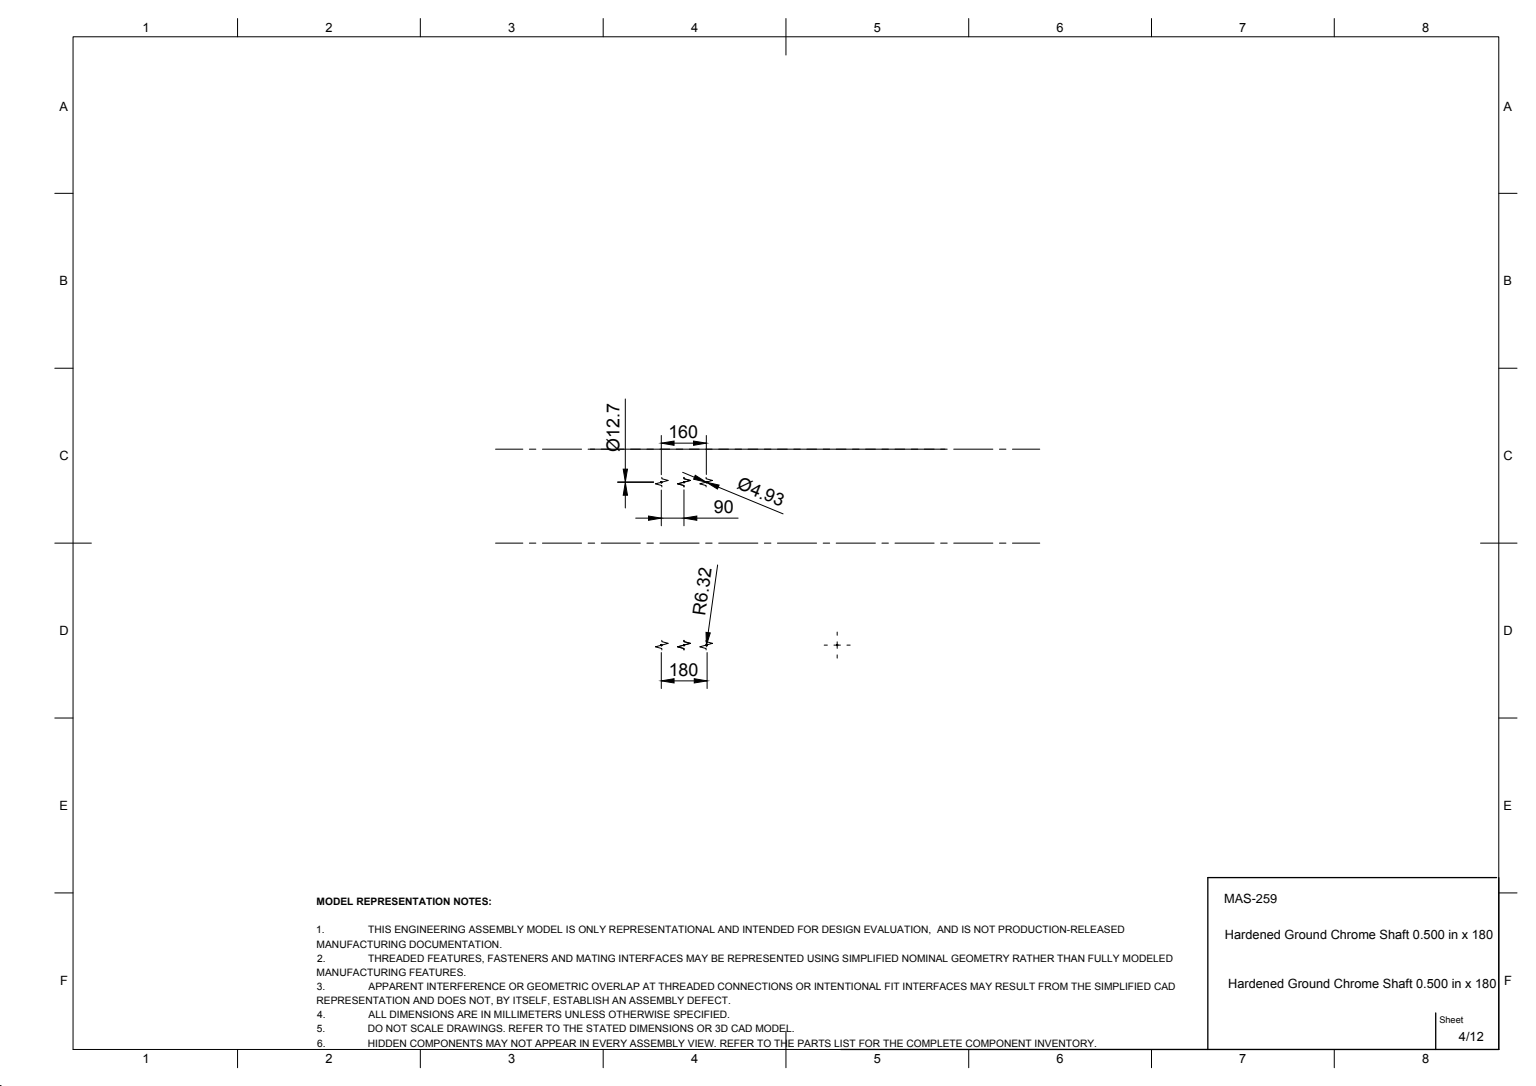
ISO-10303-21;
HEADER;
/* Generated by software containing ST-Developer
 * from STEP Tools, Inc. (www.steptools.com) 
 */

FILE_DESCRIPTION(
/* description */ (''),
/* implementation_level */ '2;1');

FILE_NAME(
/* name */ 'Hardened Ground Chrome Shaft 0.500 in x 180.step',
/* time_stamp */ '2026-10-15T13:30:17-07:00',
/* author */ (''),
/* organization */ (''),
/* preprocessor_version */ 'ST-DEVELOPER v20.2',
/* originating_system */ 'Autodesk Translation Framework v15.15.0.0',
/* authorisation */ '');

FILE_SCHEMA (('AUTOMOTIVE_DESIGN { 1 0 10303 214 3 1 1 }'));
ENDSEC;

DATA;
#10=MECHANICAL_DESIGN_GEOMETRIC_PRESENTATION_REPRESENTATION('',(#1035),#71795);
#1015=SHAPE_REPRESENTATION_RELATIONSHIP('SRR','None',#72019,#1025);
#1025=ADVANCED_BREP_SHAPE_REPRESENTATION('',(#1045),#71787);
#1035=STYLED_ITEM('',(#72078),#1045);
#1045=MANIFOLD_SOLID_BREP('Body1',#13637);
#1081=CONICAL_SURFACE('',#13996,2.464,1.02395598729616);
#1082=CONICAL_SURFACE('',#13999,2.464,1.02395598729616);
#1083=CONICAL_SURFACE('',#14002,2.464,1.02395598729616);
#1084=CONICAL_SURFACE('',#14005,6.1,0.785398163397447);
#1085=CONICAL_SURFACE('',#14009,6.1,0.785398163397439);
#1131=B_SPLINE_CURVE_WITH_KNOTS('',3,(#19389,#19390,#19391,#19392,#19393,
#19394,#19395,#19396,#19397,#19398,#19399,#19400,#19401,#19402,#19403,#19404,
#19405,#19406),.UNSPECIFIED.,.F.,.F.,(4,2,2,2,2,2,2,2,4),(0.,0.0939363144605702,
0.18787262892114,0.281725618013245,0.37557860710535,0.469431596197455,0.563284585289559,
0.657220899750131,0.751157214210703),.UNSPECIFIED.);
#1132=B_SPLINE_CURVE_WITH_KNOTS('',3,(#19407,#19408,#19409,#19410,#19411,
#19412,#19413,#19414,#19415,#19416,#19417,#19418,#19419,#19420,#19421,#19422,
#19423,#19424),.UNSPECIFIED.,.F.,.F.,(4,2,2,2,2,2,2,2,4),(0.751157214210703,
0.845093528671274,0.939029843131846,1.03288283222395,1.12673582131605,1.22058881040816,
1.31444179950026,1.40837811396083,1.50231442842141),.UNSPECIFIED.);
#1133=B_SPLINE_CURVE_WITH_KNOTS('',3,(#19434,#19435,#19436,#19437,#19438,
#19439,#19440,#19441,#19442,#19443,#19444,#19445,#19446,#19447,#19448,#19449,
#19450,#19451),.UNSPECIFIED.,.F.,.F.,(4,2,2,2,2,2,2,2,4),(0.,0.0939363144605709,
0.187872628921142,0.281725618013246,0.375578607105351,0.469431596197456,
0.56328458528956,0.657220899750131,0.751157214210702),.UNSPECIFIED.);
#1134=B_SPLINE_CURVE_WITH_KNOTS('',3,(#19452,#19453,#19454,#19455,#19456,
#19457,#19458,#19459,#19460,#19461,#19462,#19463,#19464,#19465,#19466,#19467,
#19468,#19469),.UNSPECIFIED.,.F.,.F.,(4,2,2,2,2,2,2,2,4),(0.751157214210702,
0.845093528671273,0.939029843131844,1.03288283222395,1.12673582131605,1.22058881040816,
1.31444179950026,1.40837811396083,1.5023144284214),.UNSPECIFIED.);
#1135=B_SPLINE_CURVE_WITH_KNOTS('',3,(#19479,#19480,#19481,#19482,#19483,
#19484,#19485,#19486,#19487,#19488,#19489,#19490,#19491,#19492,#19493,#19494,
#19495,#19496),.UNSPECIFIED.,.F.,.F.,(4,2,2,2,2,2,2,2,4),(0.,0.0939363144605713,
0.187872628921143,0.281725618013247,0.375578607105351,0.469431596197456,
0.56328458528956,0.657220899750132,0.751157214210703),.UNSPECIFIED.);
#1136=B_SPLINE_CURVE_WITH_KNOTS('',3,(#19497,#19498,#19499,#19500,#19501,
#19502,#19503,#19504,#19505,#19506,#19507,#19508,#19509,#19510,#19511,#19512,
#19513,#19514),.UNSPECIFIED.,.F.,.F.,(4,2,2,2,2,2,2,2,4),(0.751157214210703,
0.845093528671273,0.939029843131844,1.03288283222395,1.12673582131605,1.22058881040816,
1.31444179950026,1.40837811396083,1.5023144284214),.UNSPECIFIED.);
#1542=FACE_BOUND('',#2862,.T.);
#1543=FACE_BOUND('',#2863,.T.);
#1544=FACE_BOUND('',#2864,.T.);
#1611=PLANE('',#14003);
#1612=PLANE('',#14011);
#2147=FACE_OUTER_BOUND('',#2853,.T.);
#2148=FACE_OUTER_BOUND('',#2854,.T.);
#2149=FACE_OUTER_BOUND('',#2855,.T.);
#2150=FACE_OUTER_BOUND('',#2856,.T.);
#2151=FACE_OUTER_BOUND('',#2857,.T.);
#2152=FACE_OUTER_BOUND('',#2858,.T.);
#2153=FACE_OUTER_BOUND('',#2859,.T.);
#2154=FACE_OUTER_BOUND('',#2860,.T.);
#2155=FACE_OUTER_BOUND('',#2861,.T.);
#2156=FACE_OUTER_BOUND('',#2865,.T.);
#2157=FACE_OUTER_BOUND('',#2866,.T.);
#2853=EDGE_LOOP('',(#9525,#9526,#9527,#9528,#9529));
#2854=EDGE_LOOP('',(#9530,#9531,#9532));
#2855=EDGE_LOOP('',(#9533,#9534,#9535,#9536,#9537));
#2856=EDGE_LOOP('',(#9538,#9539,#9540));
#2857=EDGE_LOOP('',(#9541,#9542,#9543,#9544,#9545));
#2858=EDGE_LOOP('',(#9546,#9547,#9548));
#2859=EDGE_LOOP('',(#9549));
#2860=EDGE_LOOP('',(#9550,#9551,#9552,#9553));
#2861=EDGE_LOOP('',(#9554,#9555,#9556,#9557));
#2862=EDGE_LOOP('',(#9558,#9559));
#2863=EDGE_LOOP('',(#9560,#9561));
#2864=EDGE_LOOP('',(#9562,#9563));
#2865=EDGE_LOOP('',(#9564,#9565,#9566,#9567));
#2866=EDGE_LOOP('',(#9568));
#3512=CIRCLE('',#13995,2.464);
#3513=CIRCLE('',#13998,2.464);
#3514=CIRCLE('',#14001,2.464);
#3515=CIRCLE('',#14004,5.85);
#3516=CIRCLE('',#14006,6.35);
#3517=CIRCLE('',#14008,6.35);
#3518=CIRCLE('',#14010,5.85);
#3976=LINE('',#19426,#4887);
#3977=LINE('',#19430,#4888);
#3978=LINE('',#19471,#4889);
#3979=LINE('',#19475,#4890);
#3980=LINE('',#19516,#4891);
#3981=LINE('',#19520,#4892);
#3982=LINE('',#19527,#4893);
#3983=LINE('',#19531,#4894);
#3984=LINE('',#19534,#4895);
#4887=VECTOR('',#15659,2.464);
#4888=VECTOR('',#15664,2.464);
#4889=VECTOR('',#15667,2.464);
#4890=VECTOR('',#15672,2.464);
#4891=VECTOR('',#15675,2.464);
#4892=VECTOR('',#15680,2.464);
#4893=VECTOR('',#15689,6.1);
#4894=VECTOR('',#15694,6.35);
#4895=VECTOR('',#15697,6.1);
#5852=VERTEX_POINT('',#19387);
#5853=VERTEX_POINT('',#19388);
#5854=VERTEX_POINT('',#19425);
#5855=VERTEX_POINT('',#19429);
#5856=VERTEX_POINT('',#19432);
#5857=VERTEX_POINT('',#19433);
#5858=VERTEX_POINT('',#19470);
#5859=VERTEX_POINT('',#19474);
#5860=VERTEX_POINT('',#19477);
#5861=VERTEX_POINT('',#19478);
#5862=VERTEX_POINT('',#19515);
#5863=VERTEX_POINT('',#19519);
#5864=VERTEX_POINT('',#19522);
#5865=VERTEX_POINT('',#19525);
#5866=VERTEX_POINT('',#19529);
#5867=VERTEX_POINT('',#19533);
#7297=EDGE_CURVE('',#5852,#5853,#1131,.T.);
#7298=EDGE_CURVE('',#5853,#5852,#1132,.T.);
#7299=EDGE_CURVE('',#5853,#5854,#3976,.T.);
#7300=EDGE_CURVE('',#5854,#5854,#3512,.T.);
#7301=EDGE_CURVE('',#5855,#5854,#3977,.T.);
#7302=EDGE_CURVE('',#5856,#5857,#1133,.T.);
#7303=EDGE_CURVE('',#5857,#5856,#1134,.T.);
#7304=EDGE_CURVE('',#5857,#5858,#3978,.T.);
#7305=EDGE_CURVE('',#5858,#5858,#3513,.T.);
#7306=EDGE_CURVE('',#5859,#5858,#3979,.T.);
#7307=EDGE_CURVE('',#5860,#5861,#1135,.T.);
#7308=EDGE_CURVE('',#5861,#5860,#1136,.T.);
#7309=EDGE_CURVE('',#5861,#5862,#3980,.T.);
#7310=EDGE_CURVE('',#5862,#5862,#3514,.T.);
#7311=EDGE_CURVE('',#5863,#5862,#3981,.T.);
#7312=EDGE_CURVE('',#5864,#5864,#3515,.T.);
#7313=EDGE_CURVE('',#5865,#5865,#3516,.T.);
#7314=EDGE_CURVE('',#5865,#5864,#3982,.T.);
#7315=EDGE_CURVE('',#5866,#5866,#3517,.T.);
#7316=EDGE_CURVE('',#5866,#5865,#3983,.T.);
#7317=EDGE_CURVE('',#5866,#5867,#3984,.T.);
#7318=EDGE_CURVE('',#5867,#5867,#3518,.T.);
#9525=ORIENTED_EDGE('',*,*,#7297,.F.);
#9526=ORIENTED_EDGE('',*,*,#7298,.F.);
#9527=ORIENTED_EDGE('',*,*,#7299,.T.);
#9528=ORIENTED_EDGE('',*,*,#7300,.T.);
#9529=ORIENTED_EDGE('',*,*,#7299,.F.);
#9530=ORIENTED_EDGE('',*,*,#7301,.T.);
#9531=ORIENTED_EDGE('',*,*,#7300,.F.);
#9532=ORIENTED_EDGE('',*,*,#7301,.F.);
#9533=ORIENTED_EDGE('',*,*,#7302,.F.);
#9534=ORIENTED_EDGE('',*,*,#7303,.F.);
#9535=ORIENTED_EDGE('',*,*,#7304,.T.);
#9536=ORIENTED_EDGE('',*,*,#7305,.T.);
#9537=ORIENTED_EDGE('',*,*,#7304,.F.);
#9538=ORIENTED_EDGE('',*,*,#7306,.T.);
#9539=ORIENTED_EDGE('',*,*,#7305,.F.);
#9540=ORIENTED_EDGE('',*,*,#7306,.F.);
#9541=ORIENTED_EDGE('',*,*,#7307,.F.);
#9542=ORIENTED_EDGE('',*,*,#7308,.F.);
#9543=ORIENTED_EDGE('',*,*,#7309,.T.);
#9544=ORIENTED_EDGE('',*,*,#7310,.T.);
#9545=ORIENTED_EDGE('',*,*,#7309,.F.);
#9546=ORIENTED_EDGE('',*,*,#7311,.T.);
#9547=ORIENTED_EDGE('',*,*,#7310,.F.);
#9548=ORIENTED_EDGE('',*,*,#7311,.F.);
#9549=ORIENTED_EDGE('',*,*,#7312,.F.);
#9550=ORIENTED_EDGE('',*,*,#7313,.F.);
#9551=ORIENTED_EDGE('',*,*,#7314,.T.);
#9552=ORIENTED_EDGE('',*,*,#7312,.T.);
#9553=ORIENTED_EDGE('',*,*,#7314,.F.);
#9554=ORIENTED_EDGE('',*,*,#7315,.F.);
#9555=ORIENTED_EDGE('',*,*,#7316,.T.);
#9556=ORIENTED_EDGE('',*,*,#7313,.T.);
#9557=ORIENTED_EDGE('',*,*,#7316,.F.);
#9558=ORIENTED_EDGE('',*,*,#7297,.T.);
#9559=ORIENTED_EDGE('',*,*,#7298,.T.);
#9560=ORIENTED_EDGE('',*,*,#7302,.T.);
#9561=ORIENTED_EDGE('',*,*,#7303,.T.);
#9562=ORIENTED_EDGE('',*,*,#7307,.T.);
#9563=ORIENTED_EDGE('',*,*,#7308,.T.);
#9564=ORIENTED_EDGE('',*,*,#7315,.T.);
#9565=ORIENTED_EDGE('',*,*,#7317,.T.);
#9566=ORIENTED_EDGE('',*,*,#7318,.F.);
#9567=ORIENTED_EDGE('',*,*,#7317,.F.);
#9568=ORIENTED_EDGE('',*,*,#7318,.T.);
#12907=CYLINDRICAL_SURFACE('',#13994,2.464);
#12908=CYLINDRICAL_SURFACE('',#13997,2.464);
#12909=CYLINDRICAL_SURFACE('',#14000,2.464);
#12910=CYLINDRICAL_SURFACE('',#14007,6.35);
#13107=ADVANCED_FACE('',(#2147),#12907,.F.);
#13108=ADVANCED_FACE('',(#2148),#1081,.F.);
#13109=ADVANCED_FACE('',(#2149),#12908,.F.);
#13110=ADVANCED_FACE('',(#2150),#1082,.F.);
#13111=ADVANCED_FACE('',(#2151),#12909,.F.);
#13112=ADVANCED_FACE('',(#2152),#1083,.F.);
#13113=ADVANCED_FACE('',(#2153),#1611,.T.);
#13114=ADVANCED_FACE('',(#2154),#1084,.T.);
#13115=ADVANCED_FACE('',(#2155,#1542,#1543,#1544),#12910,.T.);
#13116=ADVANCED_FACE('',(#2156),#1085,.T.);
#13117=ADVANCED_FACE('',(#2157),#1612,.T.);
#13637=CLOSED_SHELL('',(#13107,#13108,#13109,#13110,#13111,#13112,#13113,
#13114,#13115,#13116,#13117));
#13993=AXIS2_PLACEMENT_3D('',#19385,#15655,#15656);
#13994=AXIS2_PLACEMENT_3D('',#19386,#15657,#15658);
#13995=AXIS2_PLACEMENT_3D('',#19427,#15660,#15661);
#13996=AXIS2_PLACEMENT_3D('',#19428,#15662,#15663);
#13997=AXIS2_PLACEMENT_3D('',#19431,#15665,#15666);
#13998=AXIS2_PLACEMENT_3D('',#19472,#15668,#15669);
#13999=AXIS2_PLACEMENT_3D('',#19473,#15670,#15671);
#14000=AXIS2_PLACEMENT_3D('',#19476,#15673,#15674);
#14001=AXIS2_PLACEMENT_3D('',#19517,#15676,#15677);
#14002=AXIS2_PLACEMENT_3D('',#19518,#15678,#15679);
#14003=AXIS2_PLACEMENT_3D('',#19521,#15681,#15682);
#14004=AXIS2_PLACEMENT_3D('',#19523,#15683,#15684);
#14005=AXIS2_PLACEMENT_3D('',#19524,#15685,#15686);
#14006=AXIS2_PLACEMENT_3D('',#19526,#15687,#15688);
#14007=AXIS2_PLACEMENT_3D('',#19528,#15690,#15691);
#14008=AXIS2_PLACEMENT_3D('',#19530,#15692,#15693);
#14009=AXIS2_PLACEMENT_3D('',#19532,#15695,#15696);
#14010=AXIS2_PLACEMENT_3D('',#19535,#15698,#15699);
#14011=AXIS2_PLACEMENT_3D('',#19536,#15700,#15701);
#15655=DIRECTION('axis',(0.,0.,1.));
#15656=DIRECTION('refdir',(1.,0.,0.));
#15657=DIRECTION('center_axis',(0.,0.707106781186548,0.707106781186548));
#15658=DIRECTION('ref_axis',(0.,-0.707106781186548,0.707106781186548));
#15659=DIRECTION('',(0.,0.707106781186548,0.707106781186548));
#15660=DIRECTION('center_axis',(0.,0.707106781186548,0.707106781186548));
#15661=DIRECTION('ref_axis',(1.,0.,0.));
#15662=DIRECTION('center_axis',(0.,-0.707106781186548,-0.707106781186548));
#15663=DIRECTION('ref_axis',(0.,-0.707106781186548,0.707106781186548));
#15664=DIRECTION('',(1.04605873377251E-16,0.236301539303659,-0.971679773651135));
#15665=DIRECTION('center_axis',(0.,0.707106781186548,0.707106781186548));
#15666=DIRECTION('ref_axis',(0.,-0.707106781186548,0.707106781186548));
#15667=DIRECTION('',(0.,0.707106781186548,0.707106781186548));
#15668=DIRECTION('center_axis',(0.,0.707106781186548,0.707106781186548));
#15669=DIRECTION('ref_axis',(1.,0.,0.));
#15670=DIRECTION('center_axis',(0.,-0.707106781186548,-0.707106781186548));
#15671=DIRECTION('ref_axis',(0.,-0.707106781186548,0.707106781186548));
#15672=DIRECTION('',(1.04605873377251E-16,0.236301539303659,-0.971679773651135));
#15673=DIRECTION('center_axis',(0.,0.707106781186548,0.707106781186548));
#15674=DIRECTION('ref_axis',(0.,-0.707106781186548,0.707106781186548));
#15675=DIRECTION('',(0.,0.707106781186548,0.707106781186548));
#15676=DIRECTION('center_axis',(0.,0.707106781186548,0.707106781186548));
#15677=DIRECTION('ref_axis',(1.,0.,0.));
#15678=DIRECTION('center_axis',(0.,-0.707106781186548,-0.707106781186548));
#15679=DIRECTION('ref_axis',(0.,-0.707106781186548,0.707106781186548));
#15680=DIRECTION('',(1.04605873377251E-16,0.236301539303659,-0.971679773651135));
#15681=DIRECTION('center_axis',(-1.,0.,0.));
#15682=DIRECTION('ref_axis',(0.,0.,1.));
#15683=DIRECTION('center_axis',(1.,0.,0.));
#15684=DIRECTION('ref_axis',(0.,0.,-1.));
#15685=DIRECTION('center_axis',(1.,0.,0.));
#15686=DIRECTION('ref_axis',(0.,1.,0.));
#15687=DIRECTION('center_axis',(1.,0.,0.));
#15688=DIRECTION('ref_axis',(0.,0.,-1.));
#15689=DIRECTION('',(-0.707106781186548,0.707106781186547,8.65956056235492E-17));
#15690=DIRECTION('center_axis',(1.,0.,0.));
#15691=DIRECTION('ref_axis',(0.,1.,0.));
#15692=DIRECTION('center_axis',(1.,0.,0.));
#15693=DIRECTION('ref_axis',(0.,0.,-1.));
#15694=DIRECTION('',(-1.,0.,0.));
#15695=DIRECTION('center_axis',(-1.,0.,0.));
#15696=DIRECTION('ref_axis',(0.,1.,0.));
#15697=DIRECTION('',(0.707106781186554,0.707106781186541,-8.65956056235485E-17));
#15698=DIRECTION('center_axis',(1.,0.,0.));
#15699=DIRECTION('ref_axis',(0.,0.,-1.));
#15700=DIRECTION('center_axis',(1.,0.,0.));
#15701=DIRECTION('ref_axis',(0.,0.,-1.));
#19385=CARTESIAN_POINT('',(0.,0.,0.));
#19386=CARTESIAN_POINT('Origin',(160.,20.386522368915,36.261522368915));
#19387=CARTESIAN_POINT('',(160.,16.3443798161838,35.7040020338711));
#19388=CARTESIAN_POINT('',(160.,19.8290020338711,32.2193798161838));
#19389=CARTESIAN_POINT('Ctrl Pts',(160.,16.3443798161838,35.7040020338711));
#19390=CARTESIAN_POINT('Ctrl Pts',(160.313121048202,16.3443798161838,35.7040020338711));
#19391=CARTESIAN_POINT('Ctrl Pts',(160.644530562725,16.3694605042293,35.639628490954));
#19392=CARTESIAN_POINT('Ctrl Pts',(161.250438810992,16.4794607587991,35.3926861336962));
#19393=CARTESIAN_POINT('Ctrl Pts',(161.525274451059,16.5655176229446,35.2114538079158));
#19394=CARTESIAN_POINT('Ctrl Pts',(161.9591552462,16.7847783338415,34.8171144138708));
#19395=CARTESIAN_POINT('Ctrl Pts',(162.148303695899,16.9331965285742,34.5767521893323));
#19396=CARTESIAN_POINT('Ctrl Pts',(162.400811747278,17.2971590391485,34.083429001318));
#19397=CARTESIAN_POINT('Ctrl Pts',(162.464,17.5136583227266,33.8310855562043));
#19398=CARTESIAN_POINT('Ctrl Pts',(162.464,17.9560855562043,33.3886583227266));
#19399=CARTESIAN_POINT('Ctrl Pts',(162.400811747278,18.208429001318,33.1721590391485));
#19400=CARTESIAN_POINT('Ctrl Pts',(162.148303695899,18.7017521893323,32.8081965285742));
#19401=CARTESIAN_POINT('Ctrl Pts',(161.9591552462,18.9421144138708,32.6597783338415));
#19402=CARTESIAN_POINT('Ctrl Pts',(161.525274451059,19.3364538079158,32.4405176229446));
#19403=CARTESIAN_POINT('Ctrl Pts',(161.250438810992,19.5176861336962,32.3544607587991));
#19404=CARTESIAN_POINT('Ctrl Pts',(160.644530562725,19.764628490954,32.2444605042293));
#19405=CARTESIAN_POINT('Ctrl Pts',(160.313121048202,19.8290020338711,32.2193798161838));
#19406=CARTESIAN_POINT('Ctrl Pts',(160.,19.8290020338711,32.2193798161838));
#19407=CARTESIAN_POINT('Ctrl Pts',(160.,19.8290020338711,32.2193798161838));
#19408=CARTESIAN_POINT('Ctrl Pts',(159.686878951798,19.8290020338711,32.2193798161838));
#19409=CARTESIAN_POINT('Ctrl Pts',(159.355469437275,19.764628490954,32.2444605042293));
#19410=CARTESIAN_POINT('Ctrl Pts',(158.749561189008,19.5176861336961,32.3544607587991));
#19411=CARTESIAN_POINT('Ctrl Pts',(158.474725548941,19.3364538079158,32.4405176229446));
#19412=CARTESIAN_POINT('Ctrl Pts',(158.0408447538,18.9421144138708,32.6597783338415));
#19413=CARTESIAN_POINT('Ctrl Pts',(157.851696304101,18.7017521893323,32.8081965285742));
#19414=CARTESIAN_POINT('Ctrl Pts',(157.599188252722,18.208429001318,33.1721590391485));
#19415=CARTESIAN_POINT('Ctrl Pts',(157.536,17.9560855562043,33.3886583227266));
#19416=CARTESIAN_POINT('Ctrl Pts',(157.536,17.5136583227266,33.8310855562043));
#19417=CARTESIAN_POINT('Ctrl Pts',(157.599188252722,17.2971590391485,34.083429001318));
#19418=CARTESIAN_POINT('Ctrl Pts',(157.851696304101,16.9331965285742,34.5767521893323));
#19419=CARTESIAN_POINT('Ctrl Pts',(158.0408447538,16.7847783338415,34.8171144138708));
#19420=CARTESIAN_POINT('Ctrl Pts',(158.474725548941,16.5655176229446,35.2114538079158));
#19421=CARTESIAN_POINT('Ctrl Pts',(158.749561189008,16.4794607587991,35.3926861336961));
#19422=CARTESIAN_POINT('Ctrl Pts',(159.355469437275,16.3694605042293,35.639628490954));
#19423=CARTESIAN_POINT('Ctrl Pts',(159.686878951798,16.3443798161838,35.7040020338711));
#19424=CARTESIAN_POINT('Ctrl Pts',(160.,16.3443798161838,35.7040020338711));
#19425=CARTESIAN_POINT('',(160.,25.1340372978015,37.5244150801141));
#19426=CARTESIAN_POINT('',(160.,22.1288334777587,34.5192112600714));
#19427=CARTESIAN_POINT('Origin',(160.,23.3917261889578,39.2667261889578));
#19428=CARTESIAN_POINT('Origin',(160.,23.3917261889578,39.2667261889578));
#19429=CARTESIAN_POINT('',(160.,24.4523863607376,40.3273863607376));
#19430=CARTESIAN_POINT('',(160.,25.1340372978015,37.5244150801141));
#19431=CARTESIAN_POINT('Origin',(90.,20.386522368915,36.261522368915));
#19432=CARTESIAN_POINT('',(90.,16.3443798161838,35.7040020338711));
#19433=CARTESIAN_POINT('',(90.,19.8290020338711,32.2193798161838));
#19434=CARTESIAN_POINT('Ctrl Pts',(90.,16.3443798161838,35.7040020338711));
#19435=CARTESIAN_POINT('Ctrl Pts',(90.3131210482019,16.3443798161838,35.7040020338711));
#19436=CARTESIAN_POINT('Ctrl Pts',(90.6445305627248,16.3694605042293,35.639628490954));
#19437=CARTESIAN_POINT('Ctrl Pts',(91.2504388109923,16.4794607587991,35.3926861336961));
#19438=CARTESIAN_POINT('Ctrl Pts',(91.525274451059,16.5655176229446,35.2114538079158));
#19439=CARTESIAN_POINT('Ctrl Pts',(91.9591552462002,16.7847783338415,34.8171144138708));
#19440=CARTESIAN_POINT('Ctrl Pts',(92.1483036958993,16.9331965285742,34.5767521893323));
#19441=CARTESIAN_POINT('Ctrl Pts',(92.4008117472775,17.2971590391485,34.0834290013181));
#19442=CARTESIAN_POINT('Ctrl Pts',(92.464,17.5136583227266,33.8310855562043));
#19443=CARTESIAN_POINT('Ctrl Pts',(92.464,17.9560855562043,33.3886583227266));
#19444=CARTESIAN_POINT('Ctrl Pts',(92.4008117472775,18.208429001318,33.1721590391485));
#19445=CARTESIAN_POINT('Ctrl Pts',(92.1483036958993,18.7017521893323,32.8081965285742));
#19446=CARTESIAN_POINT('Ctrl Pts',(91.9591552462002,18.9421144138708,32.6597783338415));
#19447=CARTESIAN_POINT('Ctrl Pts',(91.525274451059,19.3364538079158,32.4405176229446));
#19448=CARTESIAN_POINT('Ctrl Pts',(91.2504388109923,19.5176861336961,32.3544607587991));
#19449=CARTESIAN_POINT('Ctrl Pts',(90.6445305627248,19.764628490954,32.2444605042293));
#19450=CARTESIAN_POINT('Ctrl Pts',(90.3131210482019,19.8290020338711,32.2193798161838));
#19451=CARTESIAN_POINT('Ctrl Pts',(90.,19.8290020338711,32.2193798161838));
#19452=CARTESIAN_POINT('Ctrl Pts',(90.,19.8290020338711,32.2193798161838));
#19453=CARTESIAN_POINT('Ctrl Pts',(89.6868789517981,19.8290020338711,32.2193798161838));
#19454=CARTESIAN_POINT('Ctrl Pts',(89.3554694372752,19.764628490954,32.2444605042293));
#19455=CARTESIAN_POINT('Ctrl Pts',(88.7495611890077,19.5176861336961,32.3544607587991));
#19456=CARTESIAN_POINT('Ctrl Pts',(88.474725548941,19.3364538079158,32.4405176229446));
#19457=CARTESIAN_POINT('Ctrl Pts',(88.0408447537999,18.9421144138708,32.6597783338415));
#19458=CARTESIAN_POINT('Ctrl Pts',(87.8516963041007,18.7017521893323,32.8081965285742));
#19459=CARTESIAN_POINT('Ctrl Pts',(87.5991882527224,18.208429001318,33.1721590391485));
#19460=CARTESIAN_POINT('Ctrl Pts',(87.536,17.9560855562043,33.3886583227266));
#19461=CARTESIAN_POINT('Ctrl Pts',(87.536,17.5136583227266,33.8310855562043));
#19462=CARTESIAN_POINT('Ctrl Pts',(87.5991882527224,17.2971590391485,34.0834290013181));
#19463=CARTESIAN_POINT('Ctrl Pts',(87.8516963041007,16.9331965285742,34.5767521893323));
#19464=CARTESIAN_POINT('Ctrl Pts',(88.0408447537999,16.7847783338415,34.8171144138708));
#19465=CARTESIAN_POINT('Ctrl Pts',(88.474725548941,16.5655176229446,35.2114538079158));
#19466=CARTESIAN_POINT('Ctrl Pts',(88.7495611890077,16.4794607587991,35.3926861336961));
#19467=CARTESIAN_POINT('Ctrl Pts',(89.3554694372752,16.3694605042293,35.639628490954));
#19468=CARTESIAN_POINT('Ctrl Pts',(89.6868789517981,16.3443798161838,35.7040020338711));
#19469=CARTESIAN_POINT('Ctrl Pts',(90.,16.3443798161838,35.7040020338711));
#19470=CARTESIAN_POINT('',(90.,25.1340372978015,37.5244150801141));
#19471=CARTESIAN_POINT('',(90.,22.1288334777587,34.5192112600714));
#19472=CARTESIAN_POINT('Origin',(90.,23.3917261889578,39.2667261889578));
#19473=CARTESIAN_POINT('Origin',(90.,23.3917261889578,39.2667261889578));
#19474=CARTESIAN_POINT('',(90.,24.4523863607376,40.3273863607376));
#19475=CARTESIAN_POINT('',(90.,25.1340372978015,37.5244150801141));
#19476=CARTESIAN_POINT('Origin',(20.,20.386522368915,36.261522368915));
#19477=CARTESIAN_POINT('',(20.,16.3443798161838,35.7040020338711));
#19478=CARTESIAN_POINT('',(20.,19.8290020338711,32.2193798161838));
#19479=CARTESIAN_POINT('Ctrl Pts',(20.,16.3443798161838,35.7040020338711));
#19480=CARTESIAN_POINT('Ctrl Pts',(20.3131210482019,16.3443798161838,35.7040020338711));
#19481=CARTESIAN_POINT('Ctrl Pts',(20.6445305627248,16.3694605042293,35.639628490954));
#19482=CARTESIAN_POINT('Ctrl Pts',(21.2504388109924,16.4794607587991,35.3926861336961));
#19483=CARTESIAN_POINT('Ctrl Pts',(21.525274451059,16.5655176229446,35.2114538079158));
#19484=CARTESIAN_POINT('Ctrl Pts',(21.9591552462002,16.7847783338415,34.8171144138708));
#19485=CARTESIAN_POINT('Ctrl Pts',(22.1483036958993,16.9331965285742,34.5767521893323));
#19486=CARTESIAN_POINT('Ctrl Pts',(22.4008117472775,17.2971590391485,34.083429001318));
#19487=CARTESIAN_POINT('Ctrl Pts',(22.464,17.5136583227266,33.8310855562043));
#19488=CARTESIAN_POINT('Ctrl Pts',(22.464,17.9560855562043,33.3886583227266));
#19489=CARTESIAN_POINT('Ctrl Pts',(22.4008117472775,18.208429001318,33.1721590391485));
#19490=CARTESIAN_POINT('Ctrl Pts',(22.1483036958993,18.7017521893323,32.8081965285742));
#19491=CARTESIAN_POINT('Ctrl Pts',(21.9591552462002,18.9421144138708,32.6597783338415));
#19492=CARTESIAN_POINT('Ctrl Pts',(21.525274451059,19.3364538079158,32.4405176229446));
#19493=CARTESIAN_POINT('Ctrl Pts',(21.2504388109924,19.5176861336961,32.3544607587991));
#19494=CARTESIAN_POINT('Ctrl Pts',(20.6445305627248,19.764628490954,32.2444605042293));
#19495=CARTESIAN_POINT('Ctrl Pts',(20.3131210482019,19.8290020338711,32.2193798161838));
#19496=CARTESIAN_POINT('Ctrl Pts',(20.,19.8290020338711,32.2193798161838));
#19497=CARTESIAN_POINT('Ctrl Pts',(20.,19.8290020338711,32.2193798161838));
#19498=CARTESIAN_POINT('Ctrl Pts',(19.6868789517981,19.8290020338711,32.2193798161838));
#19499=CARTESIAN_POINT('Ctrl Pts',(19.3554694372752,19.764628490954,32.2444605042293));
#19500=CARTESIAN_POINT('Ctrl Pts',(18.7495611890077,19.5176861336961,32.3544607587991));
#19501=CARTESIAN_POINT('Ctrl Pts',(18.474725548941,19.3364538079158,32.4405176229446));
#19502=CARTESIAN_POINT('Ctrl Pts',(18.0408447537999,18.9421144138708,32.6597783338415));
#19503=CARTESIAN_POINT('Ctrl Pts',(17.8516963041007,18.7017521893323,32.8081965285742));
#19504=CARTESIAN_POINT('Ctrl Pts',(17.5991882527225,18.208429001318,33.1721590391485));
#19505=CARTESIAN_POINT('Ctrl Pts',(17.536,17.9560855562043,33.3886583227266));
#19506=CARTESIAN_POINT('Ctrl Pts',(17.536,17.5136583227266,33.8310855562043));
#19507=CARTESIAN_POINT('Ctrl Pts',(17.5991882527225,17.2971590391485,34.0834290013181));
#19508=CARTESIAN_POINT('Ctrl Pts',(17.8516963041007,16.9331965285742,34.5767521893323));
#19509=CARTESIAN_POINT('Ctrl Pts',(18.0408447537999,16.7847783338415,34.8171144138708));
#19510=CARTESIAN_POINT('Ctrl Pts',(18.474725548941,16.5655176229446,35.2114538079158));
#19511=CARTESIAN_POINT('Ctrl Pts',(18.7495611890077,16.4794607587991,35.3926861336961));
#19512=CARTESIAN_POINT('Ctrl Pts',(19.3554694372752,16.3694605042293,35.639628490954));
#19513=CARTESIAN_POINT('Ctrl Pts',(19.6868789517981,16.3443798161838,35.7040020338711));
#19514=CARTESIAN_POINT('Ctrl Pts',(20.,16.3443798161838,35.7040020338711));
#19515=CARTESIAN_POINT('',(20.,25.1340372978015,37.5244150801141));
#19516=CARTESIAN_POINT('',(20.,22.1288334777587,34.5192112600714));
#19517=CARTESIAN_POINT('Origin',(20.,23.3917261889578,39.2667261889578));
#19518=CARTESIAN_POINT('Origin',(20.,23.3917261889578,39.2667261889578));
#19519=CARTESIAN_POINT('',(20.,24.4523863607376,40.3273863607376));
#19520=CARTESIAN_POINT('',(20.,25.1340372978015,37.5244150801141));
#19521=CARTESIAN_POINT('Origin',(0.,28.075,38.1));
#19522=CARTESIAN_POINT('',(-7.25114412958305E-15,16.375,38.1));
#19523=CARTESIAN_POINT('Origin',(0.,22.225,38.1));
#19524=CARTESIAN_POINT('Origin',(0.249999999999986,22.225,38.1));
#19525=CARTESIAN_POINT('',(0.499999999999999,15.875,38.1));
#19526=CARTESIAN_POINT('Origin',(0.500000000000007,22.225,38.1));
#19527=CARTESIAN_POINT('',(0.249999999999986,16.125,38.1));
#19528=CARTESIAN_POINT('Origin',(90.,22.225,38.1));
#19529=CARTESIAN_POINT('',(179.5,15.875,38.1));
#19530=CARTESIAN_POINT('Origin',(179.5,22.225,38.1));
#19531=CARTESIAN_POINT('',(90.,15.875,38.1));
#19532=CARTESIAN_POINT('Origin',(179.75,22.225,38.1));
#19533=CARTESIAN_POINT('',(180.,16.375,38.1));
#19534=CARTESIAN_POINT('',(179.75,16.125,38.1));
#19535=CARTESIAN_POINT('Origin',(180.,22.225,38.1));
#19536=CARTESIAN_POINT('Origin',(180.,22.225,38.1));
#71775=UNCERTAINTY_MEASURE_WITH_UNIT(LENGTH_MEASURE(0.01),#71796,
'DISTANCE_ACCURACY_VALUE',
'Maximum model space distance between geometric entities at asserted c
onnectivities');
#71783=UNCERTAINTY_MEASURE_WITH_UNIT(LENGTH_MEASURE(0.01),#71796,
'DISTANCE_ACCURACY_VALUE',
'Maximum model space distance between geometric entities at asserted c
onnectivities');
#71787=(
GEOMETRIC_REPRESENTATION_CONTEXT(3)
GLOBAL_UNCERTAINTY_ASSIGNED_CONTEXT((#71775))
GLOBAL_UNIT_ASSIGNED_CONTEXT((#71796,#71798,#71799))
REPRESENTATION_CONTEXT('','3D')
);
#71795=(
GEOMETRIC_REPRESENTATION_CONTEXT(3)
GLOBAL_UNCERTAINTY_ASSIGNED_CONTEXT((#71783))
GLOBAL_UNIT_ASSIGNED_CONTEXT((#71796,#71798,#71799))
REPRESENTATION_CONTEXT('','3D')
);
#71796=(
LENGTH_UNIT()
NAMED_UNIT(*)
SI_UNIT(.MILLI.,.METRE.)
);
#71798=(
NAMED_UNIT(*)
PLANE_ANGLE_UNIT()
SI_UNIT($,.RADIAN.)
);
#71799=(
NAMED_UNIT(*)
SI_UNIT($,.STERADIAN.)
SOLID_ANGLE_UNIT()
);
#71803=SHAPE_DEFINITION_REPRESENTATION(#71814,#72019);
#71814=PRODUCT_DEFINITION_SHAPE('',$,#72031);
#72019=SHAPE_REPRESENTATION('',(#13993),#71787);
#72027=PRODUCT_DEFINITION_CONTEXT('part definition',#72062,'design');
#72031=PRODUCT_DEFINITION('Hardened Ground Chrome Shaft 0.500 in x 180',
'Hardened Ground Chrome Shaft 0.500 in x 180',#72042,#72027);
#72042=PRODUCT_DEFINITION_FORMATION('',$,#72067);
#72062=APPLICATION_CONTEXT(
'Core Data for Automotive Mechanical Design Process');
#72063=PRODUCT_CONTEXT('part definition',#72062,'mechanical');
#72067=PRODUCT('Hardened Ground Chrome Shaft 0.500 in x 180',
'Hardened Ground Chrome Shaft 0.500 in x 180',$,(#72063));
#72078=PRESENTATION_STYLE_ASSIGNMENT((#72089));
#72089=SURFACE_STYLE_USAGE(.BOTH.,#72100);
#72100=SURFACE_SIDE_STYLE('',(#72111));
#72111=SURFACE_STYLE_FILL_AREA(#72122);
#72122=FILL_AREA_STYLE('Opaque(236,238,241)',(#72133));
#72133=FILL_AREA_STYLE_COLOUR('Opaque(236,238,241)',#72144);
#72144=COLOUR_RGB('Opaque(236,238,241)', 0.31764706, 0.68627451, 0.89019608);
ENDSEC;
END-ISO-10303-21;
